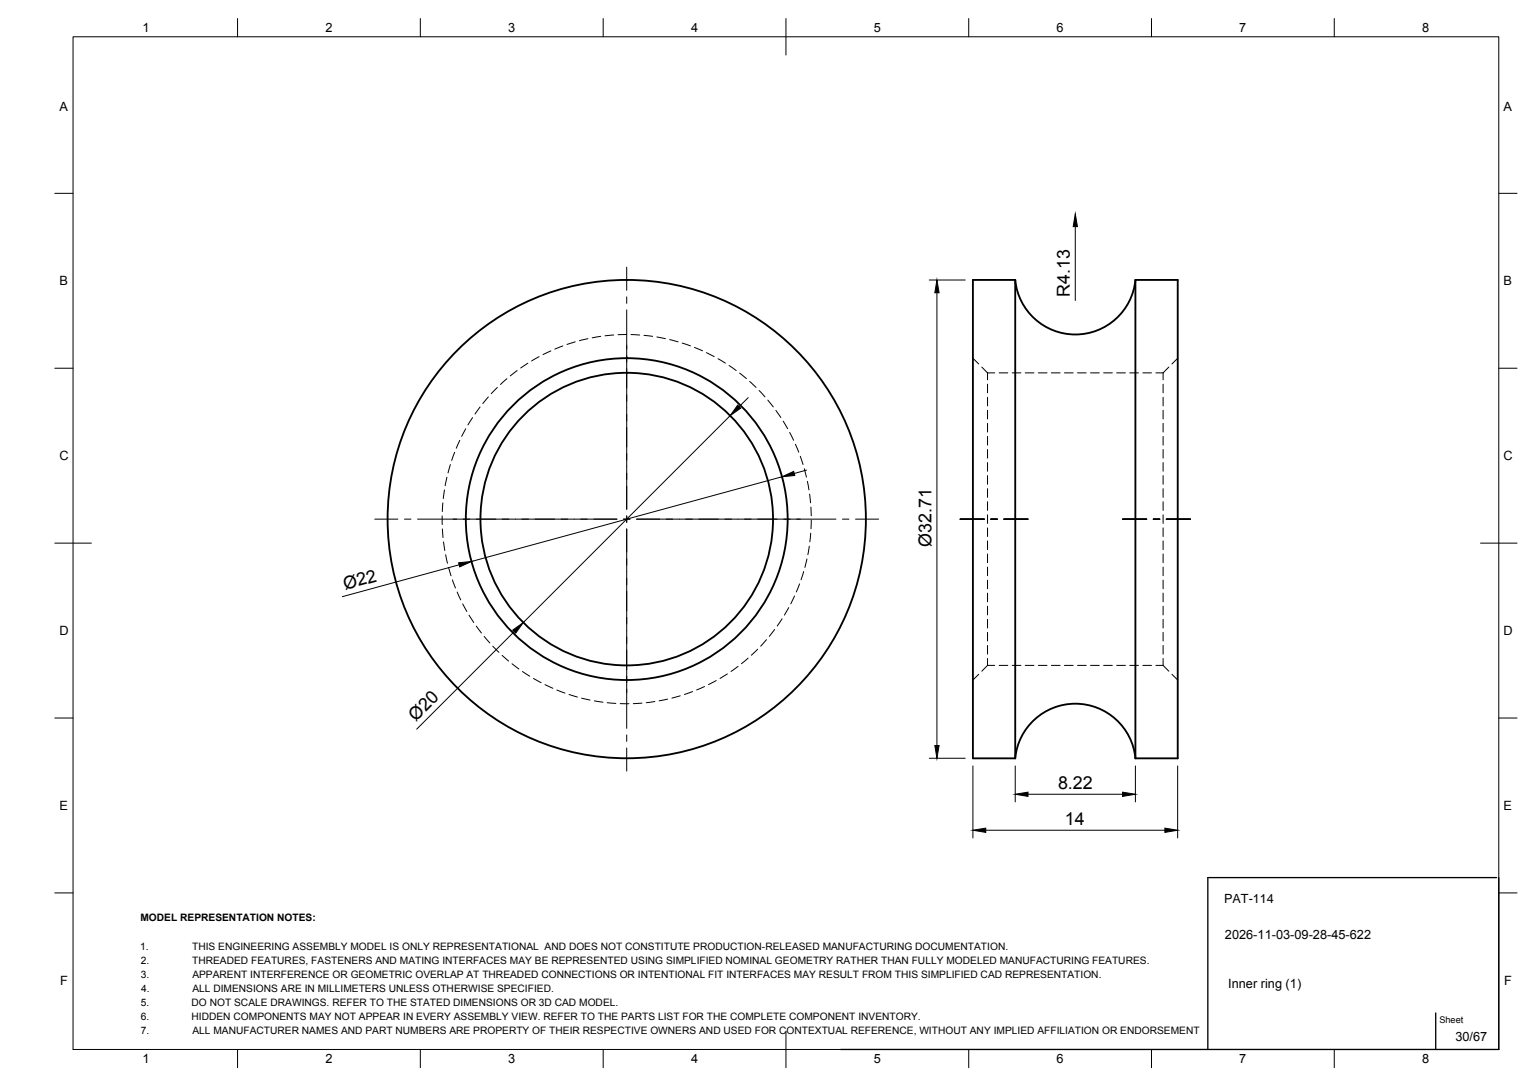
ISO-10303-21;
HEADER;
/* Generated by software containing ST-Developer
 * from STEP Tools, Inc. (www.steptools.com) 
 */

FILE_DESCRIPTION(
/* description */ ('Two-stage gear reducer in split housing'),
/* implementation_level */ '2;1');

FILE_NAME(
/* name */ 'Inner ring (1).step',
/* time_stamp */ '2026-10-28T03:22:31-07:00',
/* author */ (''),
/* organization */ (''),
/* preprocessor_version */ 'ST-DEVELOPER v20.2',
/* originating_system */ 'Autodesk Translation Framework v15.17.0.0',
/* authorisation */ '');

FILE_SCHEMA (('AUTOMOTIVE_DESIGN { 1 0 10303 214 3 1 1 }'));
ENDSEC;

DATA;
#10=MECHANICAL_DESIGN_GEOMETRIC_PRESENTATION_REPRESENTATION('',(#1263),#73366);
#1099=TOROIDAL_SURFACE('',#17546,1.675,0.412776);
#1108=CONICAL_SURFACE('',#17557,1.05,0.785398163397449);
#1109=CONICAL_SURFACE('',#17564,1.05,0.785398163397449);
#1144=SHAPE_REPRESENTATION_RELATIONSHIP('SRR','None',#73633,#1200);
#1200=ADVANCED_BREP_SHAPE_REPRESENTATION('',(#1333),#73329);
#1263=STYLED_ITEM('',(#73988),#1333);
#1333=MANIFOLD_SOLID_BREP('Body1',#16152);
#1528=FACE_BOUND('',#3420,.T.);
#1529=FACE_BOUND('',#3423,.T.);
#1771=PLANE('',#17559);
#1772=PLANE('',#17562);
#2348=FACE_OUTER_BOUND('',#3415,.T.);
#2349=FACE_OUTER_BOUND('',#3416,.T.);
#2350=FACE_OUTER_BOUND('',#3417,.T.);
#2351=FACE_OUTER_BOUND('',#3418,.T.);
#2352=FACE_OUTER_BOUND('',#3419,.T.);
#2353=FACE_OUTER_BOUND('',#3421,.T.);
#2354=FACE_OUTER_BOUND('',#3422,.T.);
#2355=FACE_OUTER_BOUND('',#3424,.T.);
#3415=EDGE_LOOP('',(#12013,#12014,#12015,#12016,#12017,#12018));
#3416=EDGE_LOOP('',(#12019,#12020,#12021,#12022,#12023));
#3417=EDGE_LOOP('',(#12024,#12025,#12026,#12027));
#3418=EDGE_LOOP('',(#12028,#12029,#12030,#12031));
#3419=EDGE_LOOP('',(#12032));
#3420=EDGE_LOOP('',(#12033));
#3421=EDGE_LOOP('',(#12034,#12035,#12036,#12037,#12038));
#3422=EDGE_LOOP('',(#12039));
#3423=EDGE_LOOP('',(#12040));
#3424=EDGE_LOOP('',(#12041,#12042,#12043,#12044));
#4439=LINE('',#24720,#5463);
#4440=LINE('',#24726,#5464);
#4441=LINE('',#24730,#5465);
#4442=LINE('',#24736,#5466);
#4443=LINE('',#24741,#5467);
#5463=VECTOR('',#20323,1.63531);
#5464=VECTOR('',#20330,1.);
#5465=VECTOR('',#20335,1.05);
#5466=VECTOR('',#20344,1.63531);
#5467=VECTOR('',#20351,1.05);
#6460=CIRCLE('',#17547,1.63531);
#6461=CIRCLE('',#17548,1.63531);
#6462=CIRCLE('',#17549,0.412776);
#6463=CIRCLE('',#17550,1.63531);
#6464=CIRCLE('',#17551,1.63531);
#6465=CIRCLE('',#17553,1.63531);
#6466=CIRCLE('',#17555,1.);
#6467=CIRCLE('',#17556,1.);
#6468=CIRCLE('',#17558,1.1);
#6469=CIRCLE('',#17561,1.63531);
#6470=CIRCLE('',#17563,1.1);
#7333=VERTEX_POINT('',#24709);
#7334=VERTEX_POINT('',#24710);
#7335=VERTEX_POINT('',#24713);
#7336=VERTEX_POINT('',#24715);
#7337=VERTEX_POINT('',#24719);
#7338=VERTEX_POINT('',#24723);
#7339=VERTEX_POINT('',#24725);
#7340=VERTEX_POINT('',#24729);
#7341=VERTEX_POINT('',#24734);
#7342=VERTEX_POINT('',#24738);
#9060=EDGE_CURVE('',#7333,#7334,#6460,.T.);
#9061=EDGE_CURVE('',#7334,#7333,#6461,.T.);
#9062=EDGE_CURVE('',#7334,#7335,#6462,.T.);
#9063=EDGE_CURVE('',#7336,#7335,#6463,.T.);
#9064=EDGE_CURVE('',#7335,#7336,#6464,.T.);
#9065=EDGE_CURVE('',#7336,#7337,#4439,.T.);
#9066=EDGE_CURVE('',#7337,#7337,#6465,.T.);
#9067=EDGE_CURVE('',#7338,#7338,#6466,.T.);
#9068=EDGE_CURVE('',#7338,#7339,#4440,.T.);
#9069=EDGE_CURVE('',#7339,#7339,#6467,.T.);
#9070=EDGE_CURVE('',#7339,#7340,#4441,.T.);
#9071=EDGE_CURVE('',#7340,#7340,#6468,.T.);
#9072=EDGE_CURVE('',#7341,#7341,#6469,.T.);
#9073=EDGE_CURVE('',#7341,#7333,#4442,.T.);
#9074=EDGE_CURVE('',#7342,#7342,#6470,.T.);
#9075=EDGE_CURVE('',#7342,#7338,#4443,.T.);
#12013=ORIENTED_EDGE('',*,*,#9060,.F.);
#12014=ORIENTED_EDGE('',*,*,#9061,.F.);
#12015=ORIENTED_EDGE('',*,*,#9062,.T.);
#12016=ORIENTED_EDGE('',*,*,#9063,.F.);
#12017=ORIENTED_EDGE('',*,*,#9064,.F.);
#12018=ORIENTED_EDGE('',*,*,#9062,.F.);
#12019=ORIENTED_EDGE('',*,*,#9063,.T.);
#12020=ORIENTED_EDGE('',*,*,#9064,.T.);
#12021=ORIENTED_EDGE('',*,*,#9065,.T.);
#12022=ORIENTED_EDGE('',*,*,#9066,.T.);
#12023=ORIENTED_EDGE('',*,*,#9065,.F.);
#12024=ORIENTED_EDGE('',*,*,#9067,.T.);
#12025=ORIENTED_EDGE('',*,*,#9068,.T.);
#12026=ORIENTED_EDGE('',*,*,#9069,.F.);
#12027=ORIENTED_EDGE('',*,*,#9068,.F.);
#12028=ORIENTED_EDGE('',*,*,#9069,.T.);
#12029=ORIENTED_EDGE('',*,*,#9070,.T.);
#12030=ORIENTED_EDGE('',*,*,#9071,.F.);
#12031=ORIENTED_EDGE('',*,*,#9070,.F.);
#12032=ORIENTED_EDGE('',*,*,#9066,.F.);
#12033=ORIENTED_EDGE('',*,*,#9071,.T.);
#12034=ORIENTED_EDGE('',*,*,#9072,.F.);
#12035=ORIENTED_EDGE('',*,*,#9073,.T.);
#12036=ORIENTED_EDGE('',*,*,#9060,.T.);
#12037=ORIENTED_EDGE('',*,*,#9061,.T.);
#12038=ORIENTED_EDGE('',*,*,#9073,.F.);
#12039=ORIENTED_EDGE('',*,*,#9072,.T.);
#12040=ORIENTED_EDGE('',*,*,#9074,.F.);
#12041=ORIENTED_EDGE('',*,*,#9074,.T.);
#12042=ORIENTED_EDGE('',*,*,#9075,.T.);
#12043=ORIENTED_EDGE('',*,*,#9067,.F.);
#12044=ORIENTED_EDGE('',*,*,#9075,.F.);
#15061=CYLINDRICAL_SURFACE('',#17552,1.63531);
#15062=CYLINDRICAL_SURFACE('',#17554,1.);
#15063=CYLINDRICAL_SURFACE('',#17560,1.63531);
#15555=ADVANCED_FACE('',(#2348),#1099,.F.);
#15556=ADVANCED_FACE('',(#2349),#15061,.T.);
#15557=ADVANCED_FACE('',(#2350),#15062,.F.);
#15558=ADVANCED_FACE('',(#2351),#1108,.F.);
#15559=ADVANCED_FACE('',(#2352,#1528),#1771,.T.);
#15560=ADVANCED_FACE('',(#2353),#15063,.T.);
#15561=ADVANCED_FACE('',(#2354,#1529),#1772,.T.);
#15562=ADVANCED_FACE('',(#2355),#1109,.F.);
#16152=CLOSED_SHELL('',(#15555,#15556,#15557,#15558,#15559,#15560,#15561,
#15562));
#17545=AXIS2_PLACEMENT_3D('',#24707,#20307,#20308);
#17546=AXIS2_PLACEMENT_3D('',#24708,#20309,#20310);
#17547=AXIS2_PLACEMENT_3D('',#24711,#20311,#20312);
#17548=AXIS2_PLACEMENT_3D('',#24712,#20313,#20314);
#17549=AXIS2_PLACEMENT_3D('',#24714,#20315,#20316);
#17550=AXIS2_PLACEMENT_3D('',#24716,#20317,#20318);
#17551=AXIS2_PLACEMENT_3D('',#24717,#20319,#20320);
#17552=AXIS2_PLACEMENT_3D('',#24718,#20321,#20322);
#17553=AXIS2_PLACEMENT_3D('',#24721,#20324,#20325);
#17554=AXIS2_PLACEMENT_3D('',#24722,#20326,#20327);
#17555=AXIS2_PLACEMENT_3D('',#24724,#20328,#20329);
#17556=AXIS2_PLACEMENT_3D('',#24727,#20331,#20332);
#17557=AXIS2_PLACEMENT_3D('',#24728,#20333,#20334);
#17558=AXIS2_PLACEMENT_3D('',#24731,#20336,#20337);
#17559=AXIS2_PLACEMENT_3D('',#24732,#20338,#20339);
#17560=AXIS2_PLACEMENT_3D('',#24733,#20340,#20341);
#17561=AXIS2_PLACEMENT_3D('',#24735,#20342,#20343);
#17562=AXIS2_PLACEMENT_3D('',#24737,#20345,#20346);
#17563=AXIS2_PLACEMENT_3D('',#24739,#20347,#20348);
#17564=AXIS2_PLACEMENT_3D('',#24740,#20349,#20350);
#20307=DIRECTION('axis',(0.,0.,1.));
#20308=DIRECTION('refdir',(1.,0.,0.));
#20309=DIRECTION('center_axis',(0.,-1.,0.));
#20310=DIRECTION('ref_axis',(0.,0.,-1.));
#20311=DIRECTION('center_axis',(0.,-1.,0.));
#20312=DIRECTION('ref_axis',(1.,0.,0.));
#20313=DIRECTION('center_axis',(0.,-1.,0.));
#20314=DIRECTION('ref_axis',(1.,0.,0.));
#20315=DIRECTION('center_axis',(1.,0.,1.22464679914735E-16));
#20316=DIRECTION('ref_axis',(-1.22464679914735E-16,0.,1.));
#20317=DIRECTION('center_axis',(0.,1.,0.));
#20318=DIRECTION('ref_axis',(1.,0.,0.));
#20319=DIRECTION('center_axis',(0.,1.,0.));
#20320=DIRECTION('ref_axis',(1.,0.,0.));
#20321=DIRECTION('center_axis',(0.,-1.,0.));
#20322=DIRECTION('ref_axis',(1.,0.,0.));
#20323=DIRECTION('',(0.,1.,0.));
#20324=DIRECTION('center_axis',(0.,-1.,0.));
#20325=DIRECTION('ref_axis',(1.,0.,0.));
#20326=DIRECTION('center_axis',(0.,-1.,0.));
#20327=DIRECTION('ref_axis',(1.,0.,0.));
#20328=DIRECTION('center_axis',(0.,-1.,0.));
#20329=DIRECTION('ref_axis',(1.,0.,0.));
#20330=DIRECTION('',(0.,1.,0.));
#20331=DIRECTION('center_axis',(0.,-1.,0.));
#20332=DIRECTION('ref_axis',(1.,0.,0.));
#20333=DIRECTION('center_axis',(0.,1.,0.));
#20334=DIRECTION('ref_axis',(1.,0.,0.));
#20335=DIRECTION('',(-0.707106781186548,0.707106781186547,-8.65956056235494E-17));
#20336=DIRECTION('center_axis',(0.,-1.,0.));
#20337=DIRECTION('ref_axis',(1.,0.,0.));
#20338=DIRECTION('center_axis',(0.,1.,0.));
#20339=DIRECTION('ref_axis',(0.,0.,1.));
#20340=DIRECTION('center_axis',(0.,-1.,0.));
#20341=DIRECTION('ref_axis',(1.,0.,0.));
#20342=DIRECTION('center_axis',(0.,-1.,0.));
#20343=DIRECTION('ref_axis',(1.,0.,0.));
#20344=DIRECTION('',(0.,1.,0.));
#20345=DIRECTION('center_axis',(0.,-1.,0.));
#20346=DIRECTION('ref_axis',(0.,0.,-1.));
#20347=DIRECTION('center_axis',(0.,-1.,0.));
#20348=DIRECTION('ref_axis',(1.,0.,0.));
#20349=DIRECTION('center_axis',(0.,-1.,0.));
#20350=DIRECTION('ref_axis',(1.,0.,0.));
#20351=DIRECTION('',(0.707106781186548,0.707106781186547,8.65956056235494E-17));
#24707=CARTESIAN_POINT('',(0.,0.,0.));
#24708=CARTESIAN_POINT('Origin',(0.,0.,0.));
#24709=CARTESIAN_POINT('',(-1.63531,-0.410863395882378,-2.00267715711366E-16));
#24710=CARTESIAN_POINT('',(-2.00267715711366E-16,-0.410863395882378,1.63531));
#24711=CARTESIAN_POINT('Origin',(0.,-0.410863395882378,0.));
#24712=CARTESIAN_POINT('Origin',(0.,-0.410863395882378,0.));
#24713=CARTESIAN_POINT('',(-2.00267715711366E-16,0.410863395882378,1.63531));
#24714=CARTESIAN_POINT('Origin',(-2.05128338857182E-16,0.,1.675));
#24715=CARTESIAN_POINT('',(-1.63531,0.410863395882378,2.00267715711366E-16));
#24716=CARTESIAN_POINT('Origin',(0.,0.410863395882378,0.));
#24717=CARTESIAN_POINT('Origin',(0.,0.410863395882378,0.));
#24718=CARTESIAN_POINT('Origin',(0.,0.,0.));
#24719=CARTESIAN_POINT('',(-1.63531,0.7,-2.00267715711366E-16));
#24720=CARTESIAN_POINT('',(-1.63531,0.,-2.00267715711366E-16));
#24721=CARTESIAN_POINT('Origin',(0.,0.7,0.));
#24722=CARTESIAN_POINT('Origin',(0.,0.,0.));
#24723=CARTESIAN_POINT('',(-1.,-0.6,-1.22464679914735E-16));
#24724=CARTESIAN_POINT('Origin',(0.,-0.6,0.));
#24725=CARTESIAN_POINT('',(-1.,0.6,-1.22464679914735E-16));
#24726=CARTESIAN_POINT('',(-1.,0.,-1.22464679914735E-16));
#24727=CARTESIAN_POINT('Origin',(0.,0.6,0.));
#24728=CARTESIAN_POINT('Origin',(0.,0.65,0.));
#24729=CARTESIAN_POINT('',(-1.1,0.7,-1.34711147906209E-16));
#24730=CARTESIAN_POINT('',(-1.05,0.65,-1.28587913910472E-16));
#24731=CARTESIAN_POINT('Origin',(0.,0.7,0.));
#24732=CARTESIAN_POINT('Origin',(1.63531,0.7,0.));
#24733=CARTESIAN_POINT('Origin',(0.,0.,0.));
#24734=CARTESIAN_POINT('',(-1.63531,-0.7,-2.00267715711366E-16));
#24735=CARTESIAN_POINT('Origin',(0.,-0.7,0.));
#24736=CARTESIAN_POINT('',(-1.63531,0.,-2.00267715711366E-16));
#24737=CARTESIAN_POINT('Origin',(1.1,-0.7,0.));
#24738=CARTESIAN_POINT('',(-1.1,-0.7,-1.34711147906209E-16));
#24739=CARTESIAN_POINT('Origin',(0.,-0.7,0.));
#24740=CARTESIAN_POINT('Origin',(0.,-0.65,0.));
#24741=CARTESIAN_POINT('',(-1.05,-0.65,-1.28587913910472E-16));
#73265=UNCERTAINTY_MEASURE_WITH_UNIT(LENGTH_MEASURE(0.001),#73367,
'DISTANCE_ACCURACY_VALUE',
'Maximum model space distance between geometric entities at asserted c
onnectivities');
#73302=UNCERTAINTY_MEASURE_WITH_UNIT(LENGTH_MEASURE(0.001),#73367,
'DISTANCE_ACCURACY_VALUE',
'Maximum model space distance between geometric entities at asserted c
onnectivities');
#73329=(
GEOMETRIC_REPRESENTATION_CONTEXT(3)
GLOBAL_UNCERTAINTY_ASSIGNED_CONTEXT((#73265))
GLOBAL_UNIT_ASSIGNED_CONTEXT((#73367,#73369,#73370))
REPRESENTATION_CONTEXT('','3D')
);
#73366=(
GEOMETRIC_REPRESENTATION_CONTEXT(3)
GLOBAL_UNCERTAINTY_ASSIGNED_CONTEXT((#73302))
GLOBAL_UNIT_ASSIGNED_CONTEXT((#73367,#73369,#73370))
REPRESENTATION_CONTEXT('','3D')
);
#73367=(
LENGTH_UNIT()
NAMED_UNIT(*)
SI_UNIT(.CENTI.,.METRE.)
);
#73369=(
NAMED_UNIT(*)
PLANE_ANGLE_UNIT()
SI_UNIT($,.RADIAN.)
);
#73370=(
NAMED_UNIT(*)
SI_UNIT($,.STERADIAN.)
SOLID_ANGLE_UNIT()
);
#73397=SHAPE_DEFINITION_REPRESENTATION(#73465,#73633);
#73465=PRODUCT_DEFINITION_SHAPE('',$,#73697);
#73633=SHAPE_REPRESENTATION('',(#17545),#73329);
#73670=PRODUCT_DEFINITION_CONTEXT('part definition',#73861,'design');
#73697=PRODUCT_DEFINITION('Inner ring (1)','Inner ring (1)',#73760,#73670);
#73760=PRODUCT_DEFINITION_FORMATION('',$,#73889);
#73861=APPLICATION_CONTEXT(
'Core Data for Automotive Mechanical Design Process');
#73862=PRODUCT_CONTEXT('part definition',#73861,'mechanical');
#73889=PRODUCT('Inner ring (1)','Inner ring (1)','Inner ring (1)',(#73862));
#73982=COLOUR_RGB('Grey',0.48,0.52,0.57);
#73983=FILL_AREA_STYLE_COLOUR('',#73982);
#73984=FILL_AREA_STYLE('',(#73983));
#73985=SURFACE_STYLE_FILL_AREA(#73984);
#73986=SURFACE_SIDE_STYLE('',(#73985));
#73987=SURFACE_STYLE_USAGE(.BOTH.,#73986);
#73988=PRESENTATION_STYLE_ASSIGNMENT((#73987));
ENDSEC;
END-ISO-10303-21;
